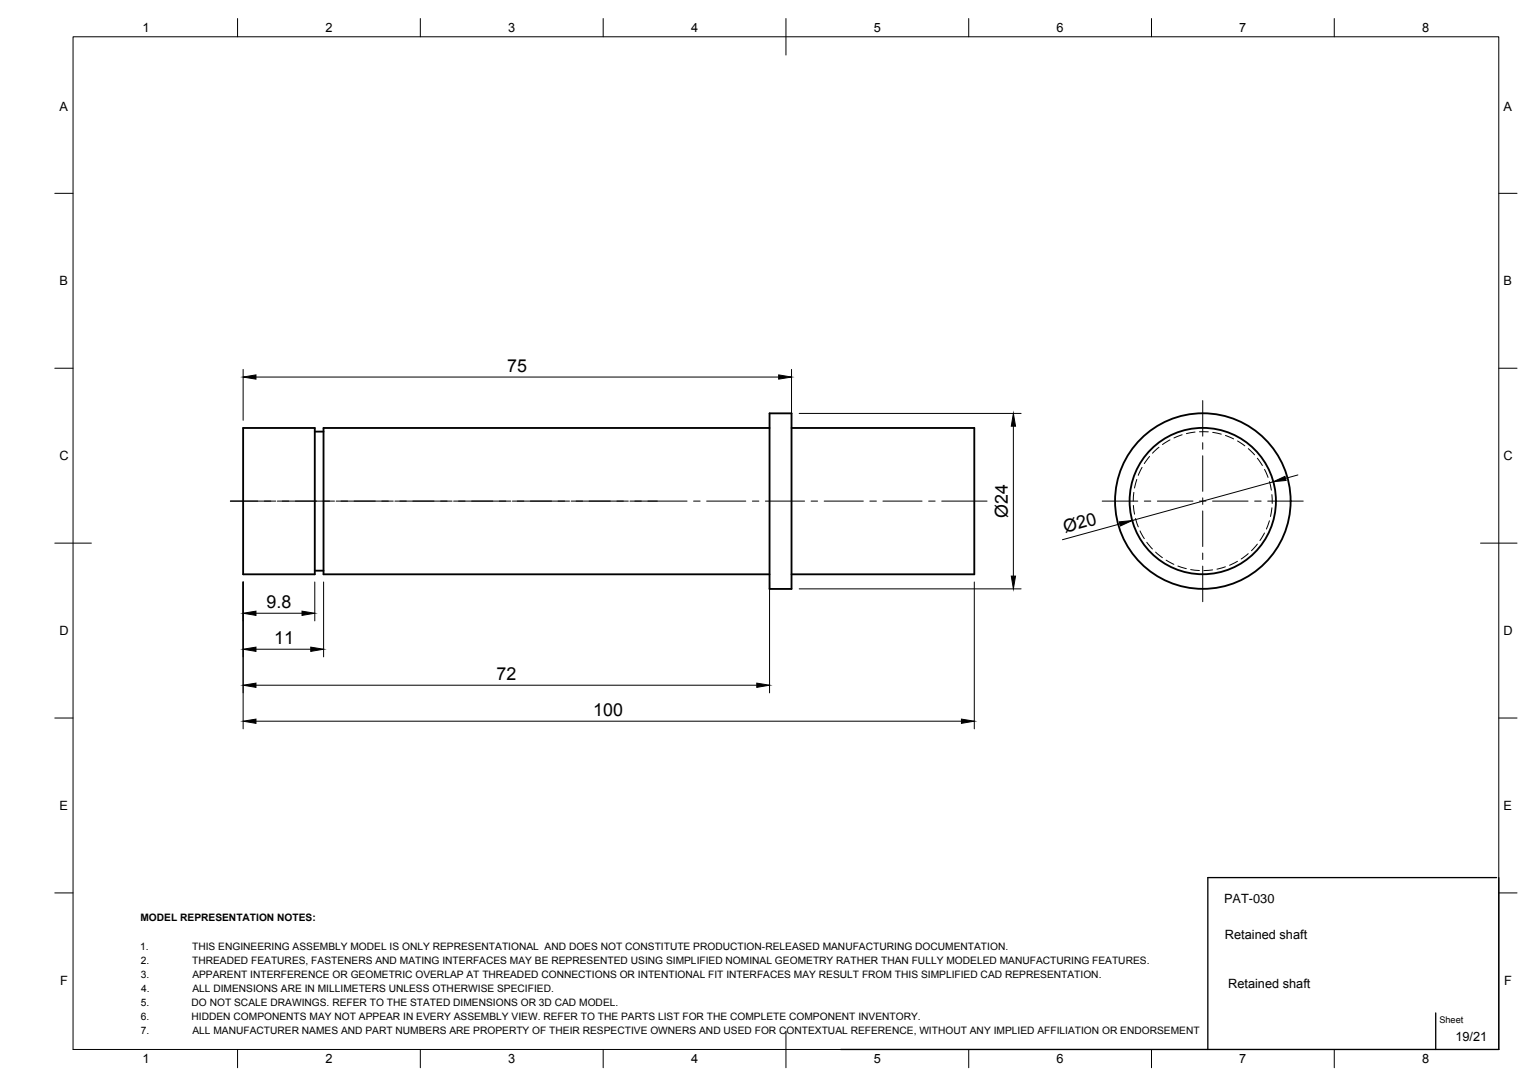
ISO-10303-21;
HEADER;
/* Generated by software containing ST-Developer
 * from STEP Tools, Inc. (www.steptools.com) 
 */

FILE_DESCRIPTION(
/* description */ ('Double-bearing flanged cartridge'),
/* implementation_level */ '2;1');

FILE_NAME(
/* name */ 'Retained shaft.step',
/* time_stamp */ '2026-10-28T03:26:40-07:00',
/* author */ (''),
/* organization */ (''),
/* preprocessor_version */ 'ST-DEVELOPER v20.2',
/* originating_system */ 'Autodesk Translation Framework v15.17.0.0',
/* authorisation */ '');

FILE_SCHEMA (('AUTOMOTIVE_DESIGN { 1 0 10303 214 3 1 1 }'));
ENDSEC;

DATA;
#10=MECHANICAL_DESIGN_GEOMETRIC_PRESENTATION_REPRESENTATION('',(#209),#5535);
#173=SHAPE_REPRESENTATION_RELATIONSHIP('SRR','None',#5616,#187);
#187=ADVANCED_BREP_SHAPE_REPRESENTATION('',(#230),#5532);
#209=STYLED_ITEM('',(#5764),#230);
#230=MANIFOLD_SOLID_BREP('Body1',#2344);
#290=FACE_BOUND('',#695,.T.);
#291=FACE_BOUND('',#697,.T.);
#292=FACE_BOUND('',#700,.T.);
#293=FACE_BOUND('',#702,.T.);
#351=PLANE('',#2817);
#352=PLANE('',#2819);
#353=PLANE('',#2823);
#354=PLANE('',#2825);
#355=PLANE('',#2833);
#356=PLANE('',#2834);
#487=FACE_OUTER_BOUND('',#693,.T.);
#488=FACE_OUTER_BOUND('',#694,.T.);
#489=FACE_OUTER_BOUND('',#696,.T.);
#490=FACE_OUTER_BOUND('',#698,.T.);
#491=FACE_OUTER_BOUND('',#699,.T.);
#492=FACE_OUTER_BOUND('',#701,.T.);
#493=FACE_OUTER_BOUND('',#703,.T.);
#494=FACE_OUTER_BOUND('',#704,.T.);
#495=FACE_OUTER_BOUND('',#705,.T.);
#496=FACE_OUTER_BOUND('',#706,.T.);
#497=FACE_OUTER_BOUND('',#707,.T.);
#693=EDGE_LOOP('',(#2036,#2037,#2038,#2039));
#694=EDGE_LOOP('',(#2040));
#695=EDGE_LOOP('',(#2041));
#696=EDGE_LOOP('',(#2042));
#697=EDGE_LOOP('',(#2043));
#698=EDGE_LOOP('',(#2044,#2045,#2046,#2047));
#699=EDGE_LOOP('',(#2048));
#700=EDGE_LOOP('',(#2049));
#701=EDGE_LOOP('',(#2050));
#702=EDGE_LOOP('',(#2051));
#703=EDGE_LOOP('',(#2052,#2053,#2054,#2055));
#704=EDGE_LOOP('',(#2056,#2057,#2058,#2059));
#705=EDGE_LOOP('',(#2060,#2061,#2062,#2063));
#706=EDGE_LOOP('',(#2064));
#707=EDGE_LOOP('',(#2065));
#801=LINE('',#4600,#887);
#802=LINE('',#4610,#888);
#803=LINE('',#4621,#889);
#804=LINE('',#4624,#890);
#805=LINE('',#4629,#891);
#887=VECTOR('',#3570,0.95);
#888=VECTOR('',#3583,1.);
#889=VECTOR('',#3598,1.2);
#890=VECTOR('',#3601,1.);
#891=VECTOR('',#3608,1.);
#1048=CIRCLE('',#2815,0.95);
#1049=CIRCLE('',#2816,0.95);
#1050=CIRCLE('',#2818,1.);
#1051=CIRCLE('',#2820,1.);
#1052=CIRCLE('',#2822,1.);
#1053=CIRCLE('',#2824,1.2);
#1054=CIRCLE('',#2826,1.2);
#1055=CIRCLE('',#2827,1.);
#1056=CIRCLE('',#2830,1.);
#1057=CIRCLE('',#2832,1.);
#1242=VERTEX_POINT('',#4597);
#1243=VERTEX_POINT('',#4599);
#1244=VERTEX_POINT('',#4603);
#1245=VERTEX_POINT('',#4606);
#1246=VERTEX_POINT('',#4609);
#1247=VERTEX_POINT('',#4613);
#1248=VERTEX_POINT('',#4616);
#1249=VERTEX_POINT('',#4618);
#1250=VERTEX_POINT('',#4623);
#1251=VERTEX_POINT('',#4627);
#1511=EDGE_CURVE('',#1242,#1242,#1048,.T.);
#1512=EDGE_CURVE('',#1242,#1243,#801,.T.);
#1513=EDGE_CURVE('',#1243,#1243,#1049,.T.);
#1514=EDGE_CURVE('',#1244,#1244,#1050,.T.);
#1515=EDGE_CURVE('',#1245,#1245,#1051,.T.);
#1516=EDGE_CURVE('',#1245,#1246,#802,.T.);
#1517=EDGE_CURVE('',#1246,#1246,#1052,.T.);
#1518=EDGE_CURVE('',#1247,#1247,#1053,.T.);
#1519=EDGE_CURVE('',#1248,#1248,#1054,.T.);
#1520=EDGE_CURVE('',#1249,#1249,#1055,.T.);
#1521=EDGE_CURVE('',#1247,#1248,#803,.T.);
#1522=EDGE_CURVE('',#1249,#1250,#804,.T.);
#1523=EDGE_CURVE('',#1250,#1250,#1056,.T.);
#1524=EDGE_CURVE('',#1251,#1251,#1057,.T.);
#1525=EDGE_CURVE('',#1251,#1244,#805,.T.);
#2036=ORIENTED_EDGE('',*,*,#1511,.F.);
#2037=ORIENTED_EDGE('',*,*,#1512,.T.);
#2038=ORIENTED_EDGE('',*,*,#1513,.T.);
#2039=ORIENTED_EDGE('',*,*,#1512,.F.);
#2040=ORIENTED_EDGE('',*,*,#1514,.F.);
#2041=ORIENTED_EDGE('',*,*,#1513,.F.);
#2042=ORIENTED_EDGE('',*,*,#1515,.F.);
#2043=ORIENTED_EDGE('',*,*,#1511,.T.);
#2044=ORIENTED_EDGE('',*,*,#1515,.T.);
#2045=ORIENTED_EDGE('',*,*,#1516,.T.);
#2046=ORIENTED_EDGE('',*,*,#1517,.T.);
#2047=ORIENTED_EDGE('',*,*,#1516,.F.);
#2048=ORIENTED_EDGE('',*,*,#1518,.T.);
#2049=ORIENTED_EDGE('',*,*,#1517,.F.);
#2050=ORIENTED_EDGE('',*,*,#1519,.F.);
#2051=ORIENTED_EDGE('',*,*,#1520,.F.);
#2052=ORIENTED_EDGE('',*,*,#1518,.F.);
#2053=ORIENTED_EDGE('',*,*,#1521,.T.);
#2054=ORIENTED_EDGE('',*,*,#1519,.T.);
#2055=ORIENTED_EDGE('',*,*,#1521,.F.);
#2056=ORIENTED_EDGE('',*,*,#1520,.T.);
#2057=ORIENTED_EDGE('',*,*,#1522,.T.);
#2058=ORIENTED_EDGE('',*,*,#1523,.T.);
#2059=ORIENTED_EDGE('',*,*,#1522,.F.);
#2060=ORIENTED_EDGE('',*,*,#1524,.F.);
#2061=ORIENTED_EDGE('',*,*,#1525,.T.);
#2062=ORIENTED_EDGE('',*,*,#1514,.T.);
#2063=ORIENTED_EDGE('',*,*,#1525,.F.);
#2064=ORIENTED_EDGE('',*,*,#1524,.T.);
#2065=ORIENTED_EDGE('',*,*,#1523,.F.);
#2163=CYLINDRICAL_SURFACE('',#2814,0.95);
#2164=CYLINDRICAL_SURFACE('',#2821,1.);
#2165=CYLINDRICAL_SURFACE('',#2828,1.2);
#2166=CYLINDRICAL_SURFACE('',#2829,1.);
#2167=CYLINDRICAL_SURFACE('',#2831,1.);
#2301=ADVANCED_FACE('',(#487),#2163,.T.);
#2302=ADVANCED_FACE('',(#488,#290),#351,.F.);
#2303=ADVANCED_FACE('',(#489,#291),#352,.T.);
#2304=ADVANCED_FACE('',(#490),#2164,.T.);
#2305=ADVANCED_FACE('',(#491,#292),#353,.T.);
#2306=ADVANCED_FACE('',(#492,#293),#354,.F.);
#2307=ADVANCED_FACE('',(#493),#2165,.T.);
#2308=ADVANCED_FACE('',(#494),#2166,.T.);
#2309=ADVANCED_FACE('',(#495),#2167,.T.);
#2310=ADVANCED_FACE('',(#496),#355,.T.);
#2311=ADVANCED_FACE('',(#497),#356,.F.);
#2344=CLOSED_SHELL('',(#2301,#2302,#2303,#2304,#2305,#2306,#2307,#2308,
#2309,#2310,#2311));
#2813=AXIS2_PLACEMENT_3D('',#4595,#3564,#3565);
#2814=AXIS2_PLACEMENT_3D('',#4596,#3566,#3567);
#2815=AXIS2_PLACEMENT_3D('',#4598,#3568,#3569);
#2816=AXIS2_PLACEMENT_3D('',#4601,#3571,#3572);
#2817=AXIS2_PLACEMENT_3D('',#4602,#3573,#3574);
#2818=AXIS2_PLACEMENT_3D('',#4604,#3575,#3576);
#2819=AXIS2_PLACEMENT_3D('',#4605,#3577,#3578);
#2820=AXIS2_PLACEMENT_3D('',#4607,#3579,#3580);
#2821=AXIS2_PLACEMENT_3D('',#4608,#3581,#3582);
#2822=AXIS2_PLACEMENT_3D('',#4611,#3584,#3585);
#2823=AXIS2_PLACEMENT_3D('',#4612,#3586,#3587);
#2824=AXIS2_PLACEMENT_3D('',#4614,#3588,#3589);
#2825=AXIS2_PLACEMENT_3D('',#4615,#3590,#3591);
#2826=AXIS2_PLACEMENT_3D('',#4617,#3592,#3593);
#2827=AXIS2_PLACEMENT_3D('',#4619,#3594,#3595);
#2828=AXIS2_PLACEMENT_3D('',#4620,#3596,#3597);
#2829=AXIS2_PLACEMENT_3D('',#4622,#3599,#3600);
#2830=AXIS2_PLACEMENT_3D('',#4625,#3602,#3603);
#2831=AXIS2_PLACEMENT_3D('',#4626,#3604,#3605);
#2832=AXIS2_PLACEMENT_3D('',#4628,#3606,#3607);
#2833=AXIS2_PLACEMENT_3D('',#4630,#3609,#3610);
#2834=AXIS2_PLACEMENT_3D('',#4631,#3611,#3612);
#3564=DIRECTION('axis',(0.,0.,1.));
#3565=DIRECTION('refdir',(1.,0.,0.));
#3566=DIRECTION('center_axis',(0.,1.,0.));
#3567=DIRECTION('ref_axis',(1.,0.,0.));
#3568=DIRECTION('center_axis',(0.,-1.,0.));
#3569=DIRECTION('ref_axis',(1.,0.,0.));
#3570=DIRECTION('',(0.,1.,0.));
#3571=DIRECTION('center_axis',(0.,-1.,0.));
#3572=DIRECTION('ref_axis',(1.,0.,0.));
#3573=DIRECTION('center_axis',(0.,1.,0.));
#3574=DIRECTION('ref_axis',(1.,0.,0.));
#3575=DIRECTION('center_axis',(0.,1.,0.));
#3576=DIRECTION('ref_axis',(1.,0.,0.));
#3577=DIRECTION('center_axis',(0.,1.,0.));
#3578=DIRECTION('ref_axis',(1.,0.,0.));
#3579=DIRECTION('center_axis',(0.,-1.,0.));
#3580=DIRECTION('ref_axis',(1.,0.,0.));
#3581=DIRECTION('center_axis',(0.,1.,0.));
#3582=DIRECTION('ref_axis',(1.,0.,0.));
#3583=DIRECTION('',(0.,-1.,0.));
#3584=DIRECTION('center_axis',(0.,1.,0.));
#3585=DIRECTION('ref_axis',(1.,0.,0.));
#3586=DIRECTION('center_axis',(0.,1.,0.));
#3587=DIRECTION('ref_axis',(1.,0.,0.));
#3588=DIRECTION('center_axis',(0.,1.,0.));
#3589=DIRECTION('ref_axis',(1.,0.,0.));
#3590=DIRECTION('center_axis',(0.,1.,0.));
#3591=DIRECTION('ref_axis',(1.,0.,0.));
#3592=DIRECTION('center_axis',(0.,1.,0.));
#3593=DIRECTION('ref_axis',(1.,0.,0.));
#3594=DIRECTION('center_axis',(0.,-1.,0.));
#3595=DIRECTION('ref_axis',(1.,0.,0.));
#3596=DIRECTION('center_axis',(0.,1.,0.));
#3597=DIRECTION('ref_axis',(1.,0.,0.));
#3598=DIRECTION('',(0.,-1.,0.));
#3599=DIRECTION('center_axis',(0.,1.,0.));
#3600=DIRECTION('ref_axis',(1.,0.,0.));
#3601=DIRECTION('',(0.,-1.,0.));
#3602=DIRECTION('center_axis',(0.,1.,0.));
#3603=DIRECTION('ref_axis',(1.,0.,0.));
#3604=DIRECTION('center_axis',(0.,1.,0.));
#3605=DIRECTION('ref_axis',(1.,0.,0.));
#3606=DIRECTION('center_axis',(0.,1.,0.));
#3607=DIRECTION('ref_axis',(1.,0.,0.));
#3608=DIRECTION('',(0.,-1.,0.));
#3609=DIRECTION('center_axis',(0.,1.,0.));
#3610=DIRECTION('ref_axis',(1.,0.,0.));
#3611=DIRECTION('center_axis',(0.,1.,0.));
#3612=DIRECTION('ref_axis',(1.,0.,0.));
#4595=CARTESIAN_POINT('',(0.,0.,0.));
#4596=CARTESIAN_POINT('Origin',(0.,6.4,4.5));
#4597=CARTESIAN_POINT('',(-0.95,6.4,4.5));
#4598=CARTESIAN_POINT('Origin',(0.,6.4,4.5));
#4599=CARTESIAN_POINT('',(-0.95,6.52,4.5));
#4600=CARTESIAN_POINT('',(-0.95,6.4,4.5));
#4601=CARTESIAN_POINT('Origin',(0.,6.52,4.5));
#4602=CARTESIAN_POINT('Origin',(0.,6.52,4.5));
#4603=CARTESIAN_POINT('',(-1.,6.52,4.5));
#4604=CARTESIAN_POINT('Origin',(0.,6.52,4.5));
#4605=CARTESIAN_POINT('Origin',(0.,6.4,4.5));
#4606=CARTESIAN_POINT('',(-1.,6.4,4.5));
#4607=CARTESIAN_POINT('Origin',(0.,6.4,4.5));
#4608=CARTESIAN_POINT('Origin',(0.,-2.5,4.5));
#4609=CARTESIAN_POINT('',(-1.,0.3,4.5));
#4610=CARTESIAN_POINT('',(-1.,-2.5,4.5));
#4611=CARTESIAN_POINT('Origin',(0.,0.3,4.5));
#4612=CARTESIAN_POINT('Origin',(0.,0.3,4.5));
#4613=CARTESIAN_POINT('',(-1.2,0.3,4.5));
#4614=CARTESIAN_POINT('Origin',(0.,0.3,4.5));
#4615=CARTESIAN_POINT('Origin',(0.,0.,4.5));
#4616=CARTESIAN_POINT('',(-1.2,0.,4.5));
#4617=CARTESIAN_POINT('Origin',(0.,0.,4.5));
#4618=CARTESIAN_POINT('',(-1.,0.,4.5));
#4619=CARTESIAN_POINT('Origin',(0.,0.,4.5));
#4620=CARTESIAN_POINT('Origin',(0.,0.,4.5));
#4621=CARTESIAN_POINT('',(-1.2,0.,4.5));
#4622=CARTESIAN_POINT('Origin',(0.,-2.5,4.5));
#4623=CARTESIAN_POINT('',(-1.,-2.5,4.5));
#4624=CARTESIAN_POINT('',(-1.,-2.5,4.5));
#4625=CARTESIAN_POINT('Origin',(0.,-2.5,4.5));
#4626=CARTESIAN_POINT('Origin',(0.,-2.5,4.5));
#4627=CARTESIAN_POINT('',(-1.,7.5,4.5));
#4628=CARTESIAN_POINT('Origin',(0.,7.5,4.5));
#4629=CARTESIAN_POINT('',(-1.,-2.5,4.5));
#4630=CARTESIAN_POINT('Origin',(0.,7.5,4.5));
#4631=CARTESIAN_POINT('Origin',(0.,-2.5,4.5));
#5513=UNCERTAINTY_MEASURE_WITH_UNIT(LENGTH_MEASURE(0.001),#5536,
'DISTANCE_ACCURACY_VALUE',
'Maximum model space distance between geometric entities at asserted c
onnectivities');
#5516=UNCERTAINTY_MEASURE_WITH_UNIT(LENGTH_MEASURE(0.001),#5536,
'DISTANCE_ACCURACY_VALUE',
'Maximum model space distance between geometric entities at asserted c
onnectivities');
#5532=(
GEOMETRIC_REPRESENTATION_CONTEXT(3)
GLOBAL_UNCERTAINTY_ASSIGNED_CONTEXT((#5513))
GLOBAL_UNIT_ASSIGNED_CONTEXT((#5536,#5538,#5539))
REPRESENTATION_CONTEXT('','3D')
);
#5535=(
GEOMETRIC_REPRESENTATION_CONTEXT(3)
GLOBAL_UNCERTAINTY_ASSIGNED_CONTEXT((#5516))
GLOBAL_UNIT_ASSIGNED_CONTEXT((#5536,#5538,#5539))
REPRESENTATION_CONTEXT('','3D')
);
#5536=(
LENGTH_UNIT()
NAMED_UNIT(*)
SI_UNIT(.CENTI.,.METRE.)
);
#5538=(
NAMED_UNIT(*)
PLANE_ANGLE_UNIT()
SI_UNIT($,.RADIAN.)
);
#5539=(
NAMED_UNIT(*)
SI_UNIT($,.STERADIAN.)
SOLID_ANGLE_UNIT()
);
#5555=SHAPE_DEFINITION_REPRESENTATION(#5593,#5616);
#5593=PRODUCT_DEFINITION_SHAPE('',$,#5635);
#5616=SHAPE_REPRESENTATION('',(#2813),#5532);
#5619=PRODUCT_DEFINITION_CONTEXT('part definition',#5675,'design');
#5635=PRODUCT_DEFINITION('Retained shaft','Retained shaft',#5653,#5619);
#5653=PRODUCT_DEFINITION_FORMATION('',$,#5692);
#5675=APPLICATION_CONTEXT(
'Core Data for Automotive Mechanical Design Process');
#5676=PRODUCT_CONTEXT('part definition',#5675,'mechanical');
#5692=PRODUCT('Retained shaft','Retained shaft','Retained shaft',(#5676));
#5758=COLOUR_RGB('Grey',0.48,0.52,0.57);
#5759=FILL_AREA_STYLE_COLOUR('',#5758);
#5760=FILL_AREA_STYLE('',(#5759));
#5761=SURFACE_STYLE_FILL_AREA(#5760);
#5762=SURFACE_SIDE_STYLE('',(#5761));
#5763=SURFACE_STYLE_USAGE(.BOTH.,#5762);
#5764=PRESENTATION_STYLE_ASSIGNMENT((#5763));
ENDSEC;
END-ISO-10303-21;
